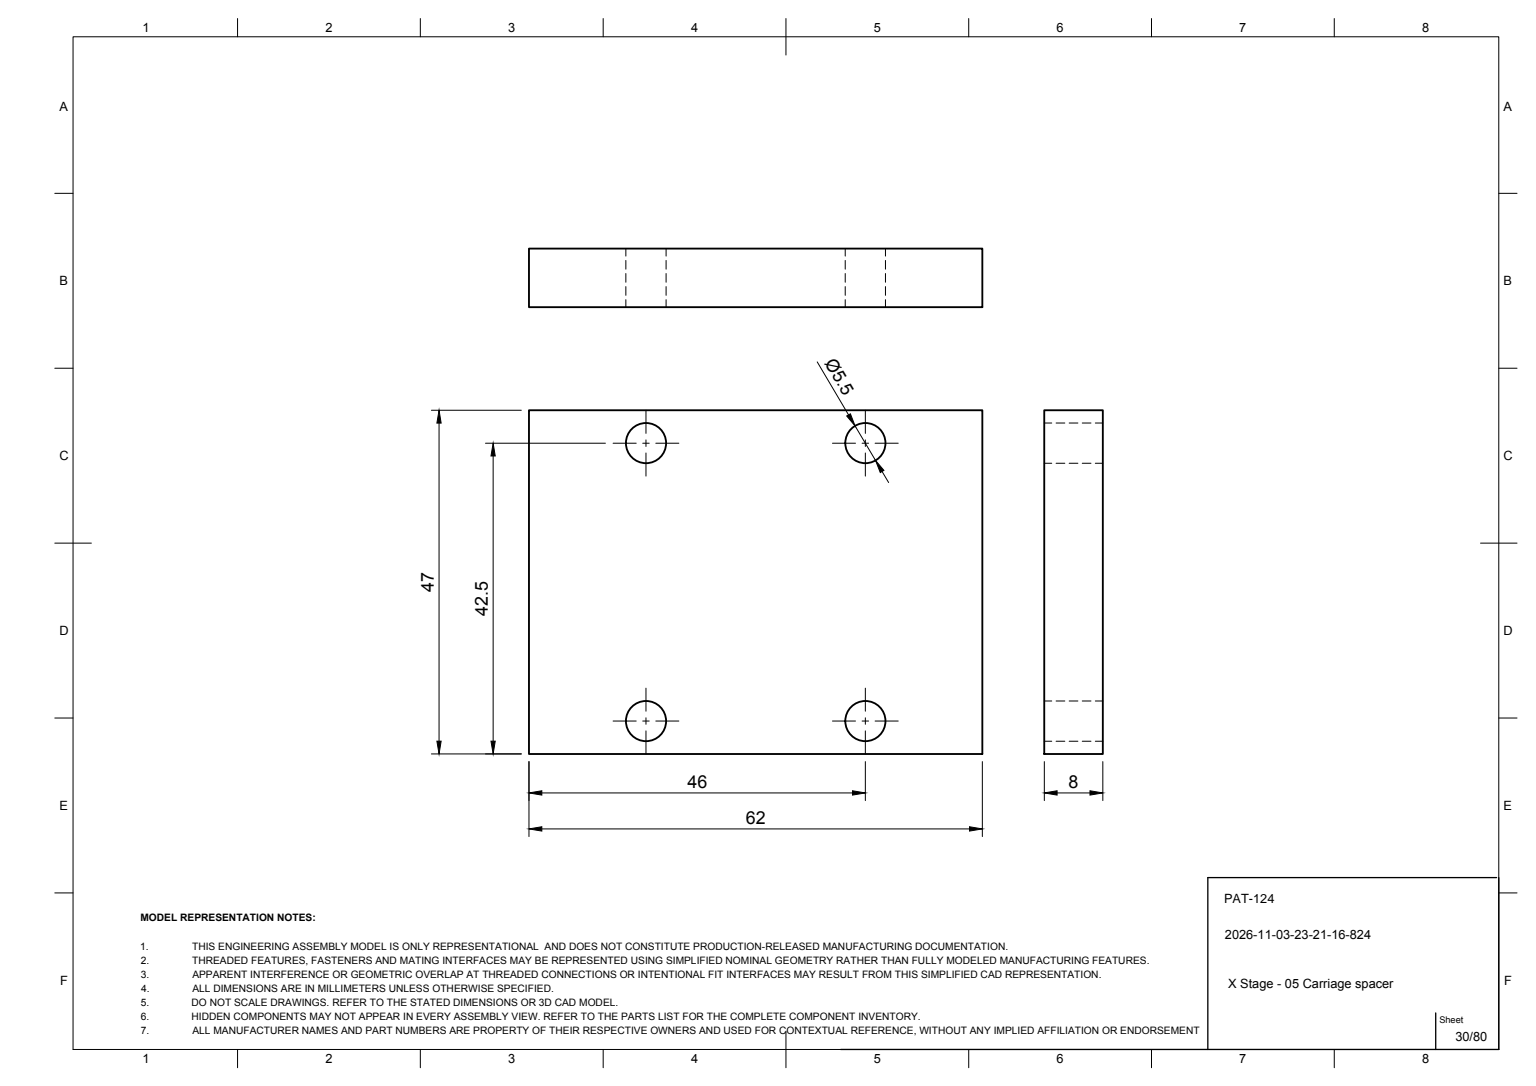
ISO-10303-21;
HEADER;
/* Generated by software containing ST-Developer
 * from STEP Tools, Inc. (www.steptools.com) 
 */

FILE_DESCRIPTION(
/* description */ ('XY cross-slide table'),
/* implementation_level */ '2;1');

FILE_NAME(
/* name */ 'X Stage - 05 Carriage spacer.step',
/* time_stamp */ '2026-10-28T03:22:46-07:00',
/* author */ (''),
/* organization */ (''),
/* preprocessor_version */ 'ST-DEVELOPER v20.2',
/* originating_system */ 'Autodesk Translation Framework v15.17.0.0',
/* authorisation */ '');

FILE_SCHEMA (('AUTOMOTIVE_DESIGN { 1 0 10303 214 3 1 1 }'));
ENDSEC;

DATA;
#10=MECHANICAL_DESIGN_GEOMETRIC_PRESENTATION_REPRESENTATION('',(#1706),#62984);
#1525=SHAPE_REPRESENTATION_RELATIONSHIP('SRR','None',#63376,#1608);
#1608=ADVANCED_BREP_SHAPE_REPRESENTATION('',(#1819),#62913);
#1706=STYLED_ITEM('',(#63898),#1819);
#1819=MANIFOLD_SOLID_BREP('Body1',#23000);
#2001=FACE_BOUND('',#4552,.T.);
#2002=FACE_BOUND('',#4553,.T.);
#2003=FACE_BOUND('',#4554,.T.);
#2004=FACE_BOUND('',#4555,.T.);
#2005=FACE_BOUND('',#4557,.T.);
#2006=FACE_BOUND('',#4558,.T.);
#2007=FACE_BOUND('',#4559,.T.);
#2008=FACE_BOUND('',#4560,.T.);
#2414=PLANE('',#24561);
#2415=PLANE('',#24562);
#2416=PLANE('',#24563);
#2417=PLANE('',#24564);
#2418=PLANE('',#24565);
#2419=PLANE('',#24566);
#3115=FACE_OUTER_BOUND('',#4543,.T.);
#3116=FACE_OUTER_BOUND('',#4544,.T.);
#3117=FACE_OUTER_BOUND('',#4545,.T.);
#3118=FACE_OUTER_BOUND('',#4546,.T.);
#3119=FACE_OUTER_BOUND('',#4547,.T.);
#3120=FACE_OUTER_BOUND('',#4548,.T.);
#3121=FACE_OUTER_BOUND('',#4549,.T.);
#3122=FACE_OUTER_BOUND('',#4550,.T.);
#3123=FACE_OUTER_BOUND('',#4551,.T.);
#3124=FACE_OUTER_BOUND('',#4556,.T.);
#4543=EDGE_LOOP('',(#15964,#15965,#15966,#15967));
#4544=EDGE_LOOP('',(#15968,#15969,#15970,#15971));
#4545=EDGE_LOOP('',(#15972,#15973,#15974,#15975));
#4546=EDGE_LOOP('',(#15976,#15977,#15978,#15979));
#4547=EDGE_LOOP('',(#15980,#15981,#15982,#15983));
#4548=EDGE_LOOP('',(#15984,#15985,#15986,#15987));
#4549=EDGE_LOOP('',(#15988,#15989,#15990,#15991));
#4550=EDGE_LOOP('',(#15992,#15993,#15994,#15995));
#4551=EDGE_LOOP('',(#15996,#15997,#15998,#15999));
#4552=EDGE_LOOP('',(#16000));
#4553=EDGE_LOOP('',(#16001));
#4554=EDGE_LOOP('',(#16002));
#4555=EDGE_LOOP('',(#16003));
#4556=EDGE_LOOP('',(#16004,#16005,#16006,#16007));
#4557=EDGE_LOOP('',(#16008));
#4558=EDGE_LOOP('',(#16009));
#4559=EDGE_LOOP('',(#16010));
#4560=EDGE_LOOP('',(#16011));
#6139=LINE('',#34688,#7626);
#6140=LINE('',#34694,#7627);
#6141=LINE('',#34700,#7628);
#6142=LINE('',#34706,#7629);
#6143=LINE('',#34711,#7630);
#6144=LINE('',#34713,#7631);
#6145=LINE('',#34715,#7632);
#6146=LINE('',#34716,#7633);
#6147=LINE('',#34719,#7634);
#6148=LINE('',#34721,#7635);
#6149=LINE('',#34722,#7636);
#6150=LINE('',#34725,#7637);
#6151=LINE('',#34727,#7638);
#6152=LINE('',#34728,#7639);
#6153=LINE('',#34730,#7640);
#6154=LINE('',#34731,#7641);
#7626=VECTOR('',#27796,0.275);
#7627=VECTOR('',#27803,0.275);
#7628=VECTOR('',#27810,0.275);
#7629=VECTOR('',#27817,0.275);
#7630=VECTOR('',#27822,1.);
#7631=VECTOR('',#27823,1.);
#7632=VECTOR('',#27824,1.);
#7633=VECTOR('',#27825,1.);
#7634=VECTOR('',#27828,1.);
#7635=VECTOR('',#27829,1.);
#7636=VECTOR('',#27830,1.);
#7637=VECTOR('',#27833,1.);
#7638=VECTOR('',#27834,1.);
#7639=VECTOR('',#27835,1.);
#7640=VECTOR('',#27838,1.);
#7641=VECTOR('',#27839,1.);
#9145=CIRCLE('',#24550,0.275);
#9146=CIRCLE('',#24551,0.275);
#9147=CIRCLE('',#24553,0.275);
#9148=CIRCLE('',#24554,0.275);
#9149=CIRCLE('',#24556,0.275);
#9150=CIRCLE('',#24557,0.275);
#9151=CIRCLE('',#24559,0.275);
#9152=CIRCLE('',#24560,0.275);
#10141=VERTEX_POINT('',#34685);
#10142=VERTEX_POINT('',#34687);
#10143=VERTEX_POINT('',#34691);
#10144=VERTEX_POINT('',#34693);
#10145=VERTEX_POINT('',#34697);
#10146=VERTEX_POINT('',#34699);
#10147=VERTEX_POINT('',#34703);
#10148=VERTEX_POINT('',#34705);
#10149=VERTEX_POINT('',#34709);
#10150=VERTEX_POINT('',#34710);
#10151=VERTEX_POINT('',#34712);
#10152=VERTEX_POINT('',#34714);
#10153=VERTEX_POINT('',#34718);
#10154=VERTEX_POINT('',#34720);
#10155=VERTEX_POINT('',#34724);
#10156=VERTEX_POINT('',#34726);
#12366=EDGE_CURVE('',#10141,#10141,#9145,.T.);
#12367=EDGE_CURVE('',#10141,#10142,#6139,.T.);
#12368=EDGE_CURVE('',#10142,#10142,#9146,.T.);
#12369=EDGE_CURVE('',#10143,#10143,#9147,.T.);
#12370=EDGE_CURVE('',#10143,#10144,#6140,.T.);
#12371=EDGE_CURVE('',#10144,#10144,#9148,.T.);
#12372=EDGE_CURVE('',#10145,#10145,#9149,.T.);
#12373=EDGE_CURVE('',#10145,#10146,#6141,.T.);
#12374=EDGE_CURVE('',#10146,#10146,#9150,.T.);
#12375=EDGE_CURVE('',#10147,#10147,#9151,.T.);
#12376=EDGE_CURVE('',#10147,#10148,#6142,.T.);
#12377=EDGE_CURVE('',#10148,#10148,#9152,.T.);
#12378=EDGE_CURVE('',#10149,#10150,#6143,.T.);
#12379=EDGE_CURVE('',#10150,#10151,#6144,.T.);
#12380=EDGE_CURVE('',#10152,#10151,#6145,.T.);
#12381=EDGE_CURVE('',#10149,#10152,#6146,.T.);
#12382=EDGE_CURVE('',#10153,#10149,#6147,.T.);
#12383=EDGE_CURVE('',#10154,#10152,#6148,.T.);
#12384=EDGE_CURVE('',#10153,#10154,#6149,.T.);
#12385=EDGE_CURVE('',#10155,#10153,#6150,.T.);
#12386=EDGE_CURVE('',#10156,#10154,#6151,.T.);
#12387=EDGE_CURVE('',#10155,#10156,#6152,.T.);
#12388=EDGE_CURVE('',#10150,#10155,#6153,.T.);
#12389=EDGE_CURVE('',#10151,#10156,#6154,.T.);
#15964=ORIENTED_EDGE('',*,*,#12366,.F.);
#15965=ORIENTED_EDGE('',*,*,#12367,.T.);
#15966=ORIENTED_EDGE('',*,*,#12368,.F.);
#15967=ORIENTED_EDGE('',*,*,#12367,.F.);
#15968=ORIENTED_EDGE('',*,*,#12369,.F.);
#15969=ORIENTED_EDGE('',*,*,#12370,.T.);
#15970=ORIENTED_EDGE('',*,*,#12371,.F.);
#15971=ORIENTED_EDGE('',*,*,#12370,.F.);
#15972=ORIENTED_EDGE('',*,*,#12372,.F.);
#15973=ORIENTED_EDGE('',*,*,#12373,.T.);
#15974=ORIENTED_EDGE('',*,*,#12374,.F.);
#15975=ORIENTED_EDGE('',*,*,#12373,.F.);
#15976=ORIENTED_EDGE('',*,*,#12375,.F.);
#15977=ORIENTED_EDGE('',*,*,#12376,.T.);
#15978=ORIENTED_EDGE('',*,*,#12377,.F.);
#15979=ORIENTED_EDGE('',*,*,#12376,.F.);
#15980=ORIENTED_EDGE('',*,*,#12378,.T.);
#15981=ORIENTED_EDGE('',*,*,#12379,.T.);
#15982=ORIENTED_EDGE('',*,*,#12380,.F.);
#15983=ORIENTED_EDGE('',*,*,#12381,.F.);
#15984=ORIENTED_EDGE('',*,*,#12382,.T.);
#15985=ORIENTED_EDGE('',*,*,#12381,.T.);
#15986=ORIENTED_EDGE('',*,*,#12383,.F.);
#15987=ORIENTED_EDGE('',*,*,#12384,.F.);
#15988=ORIENTED_EDGE('',*,*,#12385,.T.);
#15989=ORIENTED_EDGE('',*,*,#12384,.T.);
#15990=ORIENTED_EDGE('',*,*,#12386,.F.);
#15991=ORIENTED_EDGE('',*,*,#12387,.F.);
#15992=ORIENTED_EDGE('',*,*,#12388,.T.);
#15993=ORIENTED_EDGE('',*,*,#12387,.T.);
#15994=ORIENTED_EDGE('',*,*,#12389,.F.);
#15995=ORIENTED_EDGE('',*,*,#12379,.F.);
#15996=ORIENTED_EDGE('',*,*,#12389,.T.);
#15997=ORIENTED_EDGE('',*,*,#12386,.T.);
#15998=ORIENTED_EDGE('',*,*,#12383,.T.);
#15999=ORIENTED_EDGE('',*,*,#12380,.T.);
#16000=ORIENTED_EDGE('',*,*,#12368,.T.);
#16001=ORIENTED_EDGE('',*,*,#12371,.T.);
#16002=ORIENTED_EDGE('',*,*,#12374,.T.);
#16003=ORIENTED_EDGE('',*,*,#12377,.T.);
#16004=ORIENTED_EDGE('',*,*,#12388,.F.);
#16005=ORIENTED_EDGE('',*,*,#12378,.F.);
#16006=ORIENTED_EDGE('',*,*,#12382,.F.);
#16007=ORIENTED_EDGE('',*,*,#12385,.F.);
#16008=ORIENTED_EDGE('',*,*,#12366,.T.);
#16009=ORIENTED_EDGE('',*,*,#12369,.T.);
#16010=ORIENTED_EDGE('',*,*,#12372,.T.);
#16011=ORIENTED_EDGE('',*,*,#12375,.T.);
#21126=CYLINDRICAL_SURFACE('',#24549,0.275);
#21127=CYLINDRICAL_SURFACE('',#24552,0.275);
#21128=CYLINDRICAL_SURFACE('',#24555,0.275);
#21129=CYLINDRICAL_SURFACE('',#24558,0.275);
#21896=ADVANCED_FACE('',(#3115),#21126,.F.);
#21897=ADVANCED_FACE('',(#3116),#21127,.F.);
#21898=ADVANCED_FACE('',(#3117),#21128,.F.);
#21899=ADVANCED_FACE('',(#3118),#21129,.F.);
#21900=ADVANCED_FACE('',(#3119),#2414,.T.);
#21901=ADVANCED_FACE('',(#3120),#2415,.T.);
#21902=ADVANCED_FACE('',(#3121),#2416,.T.);
#21903=ADVANCED_FACE('',(#3122),#2417,.T.);
#21904=ADVANCED_FACE('',(#3123,#2001,#2002,#2003,#2004),#2418,.T.);
#21905=ADVANCED_FACE('',(#3124,#2005,#2006,#2007,#2008),#2419,.F.);
#23000=CLOSED_SHELL('',(#21896,#21897,#21898,#21899,#21900,#21901,#21902,
#21903,#21904,#21905));
#24548=AXIS2_PLACEMENT_3D('',#34683,#27790,#27791);
#24549=AXIS2_PLACEMENT_3D('',#34684,#27792,#27793);
#24550=AXIS2_PLACEMENT_3D('',#34686,#27794,#27795);
#24551=AXIS2_PLACEMENT_3D('',#34689,#27797,#27798);
#24552=AXIS2_PLACEMENT_3D('',#34690,#27799,#27800);
#24553=AXIS2_PLACEMENT_3D('',#34692,#27801,#27802);
#24554=AXIS2_PLACEMENT_3D('',#34695,#27804,#27805);
#24555=AXIS2_PLACEMENT_3D('',#34696,#27806,#27807);
#24556=AXIS2_PLACEMENT_3D('',#34698,#27808,#27809);
#24557=AXIS2_PLACEMENT_3D('',#34701,#27811,#27812);
#24558=AXIS2_PLACEMENT_3D('',#34702,#27813,#27814);
#24559=AXIS2_PLACEMENT_3D('',#34704,#27815,#27816);
#24560=AXIS2_PLACEMENT_3D('',#34707,#27818,#27819);
#24561=AXIS2_PLACEMENT_3D('',#34708,#27820,#27821);
#24562=AXIS2_PLACEMENT_3D('',#34717,#27826,#27827);
#24563=AXIS2_PLACEMENT_3D('',#34723,#27831,#27832);
#24564=AXIS2_PLACEMENT_3D('',#34729,#27836,#27837);
#24565=AXIS2_PLACEMENT_3D('',#34732,#27840,#27841);
#24566=AXIS2_PLACEMENT_3D('',#34733,#27842,#27843);
#27790=DIRECTION('axis',(0.,0.,1.));
#27791=DIRECTION('refdir',(1.,0.,0.));
#27792=DIRECTION('center_axis',(0.,0.,1.));
#27793=DIRECTION('ref_axis',(1.,0.,0.));
#27794=DIRECTION('center_axis',(0.,0.,1.));
#27795=DIRECTION('ref_axis',(1.,0.,0.));
#27796=DIRECTION('',(0.,0.,1.));
#27797=DIRECTION('center_axis',(0.,0.,-1.));
#27798=DIRECTION('ref_axis',(1.,0.,0.));
#27799=DIRECTION('center_axis',(0.,0.,1.));
#27800=DIRECTION('ref_axis',(1.,0.,0.));
#27801=DIRECTION('center_axis',(0.,0.,1.));
#27802=DIRECTION('ref_axis',(1.,0.,0.));
#27803=DIRECTION('',(0.,0.,1.));
#27804=DIRECTION('center_axis',(0.,0.,-1.));
#27805=DIRECTION('ref_axis',(1.,0.,0.));
#27806=DIRECTION('center_axis',(0.,0.,1.));
#27807=DIRECTION('ref_axis',(1.,0.,0.));
#27808=DIRECTION('center_axis',(0.,0.,1.));
#27809=DIRECTION('ref_axis',(1.,0.,0.));
#27810=DIRECTION('',(0.,0.,1.));
#27811=DIRECTION('center_axis',(0.,0.,-1.));
#27812=DIRECTION('ref_axis',(1.,0.,0.));
#27813=DIRECTION('center_axis',(0.,0.,1.));
#27814=DIRECTION('ref_axis',(1.,0.,0.));
#27815=DIRECTION('center_axis',(0.,0.,1.));
#27816=DIRECTION('ref_axis',(1.,0.,0.));
#27817=DIRECTION('',(0.,0.,1.));
#27818=DIRECTION('center_axis',(0.,0.,-1.));
#27819=DIRECTION('ref_axis',(1.,0.,0.));
#27820=DIRECTION('center_axis',(0.,1.,0.));
#27821=DIRECTION('ref_axis',(-1.,0.,0.));
#27822=DIRECTION('',(-1.,0.,0.));
#27823=DIRECTION('',(0.,0.,1.));
#27824=DIRECTION('',(-1.,0.,0.));
#27825=DIRECTION('',(0.,0.,1.));
#27826=DIRECTION('center_axis',(1.,0.,0.));
#27827=DIRECTION('ref_axis',(0.,1.,0.));
#27828=DIRECTION('',(0.,1.,0.));
#27829=DIRECTION('',(0.,1.,0.));
#27830=DIRECTION('',(0.,0.,1.));
#27831=DIRECTION('center_axis',(0.,-1.,0.));
#27832=DIRECTION('ref_axis',(1.,0.,0.));
#27833=DIRECTION('',(1.,0.,0.));
#27834=DIRECTION('',(1.,0.,0.));
#27835=DIRECTION('',(0.,0.,1.));
#27836=DIRECTION('center_axis',(-1.,0.,0.));
#27837=DIRECTION('ref_axis',(0.,-1.,0.));
#27838=DIRECTION('',(0.,-1.,0.));
#27839=DIRECTION('',(0.,-1.,0.));
#27840=DIRECTION('center_axis',(0.,0.,1.));
#27841=DIRECTION('ref_axis',(1.,0.,0.));
#27842=DIRECTION('center_axis',(0.,0.,1.));
#27843=DIRECTION('ref_axis',(1.,0.,0.));
#34683=CARTESIAN_POINT('',(0.,0.,0.));
#34684=CARTESIAN_POINT('Origin',(15.,-7.9,5.1));
#34685=CARTESIAN_POINT('',(14.725,-7.9,5.2));
#34686=CARTESIAN_POINT('Origin',(15.,-7.9,5.2));
#34687=CARTESIAN_POINT('',(14.725,-7.9,6.));
#34688=CARTESIAN_POINT('',(14.725,-7.9,5.1));
#34689=CARTESIAN_POINT('Origin',(15.,-7.9,6.));
#34690=CARTESIAN_POINT('Origin',(12.,-4.1,5.1));
#34691=CARTESIAN_POINT('',(11.725,-4.1,5.2));
#34692=CARTESIAN_POINT('Origin',(12.,-4.1,5.2));
#34693=CARTESIAN_POINT('',(11.725,-4.1,6.));
#34694=CARTESIAN_POINT('',(11.725,-4.1,5.1));
#34695=CARTESIAN_POINT('Origin',(12.,-4.1,6.));
#34696=CARTESIAN_POINT('Origin',(12.,-7.9,5.1));
#34697=CARTESIAN_POINT('',(11.725,-7.9,5.2));
#34698=CARTESIAN_POINT('Origin',(12.,-7.9,5.2));
#34699=CARTESIAN_POINT('',(11.725,-7.9,6.));
#34700=CARTESIAN_POINT('',(11.725,-7.9,5.1));
#34701=CARTESIAN_POINT('Origin',(12.,-7.9,6.));
#34702=CARTESIAN_POINT('Origin',(15.,-4.1,5.1));
#34703=CARTESIAN_POINT('',(14.725,-4.1,5.2));
#34704=CARTESIAN_POINT('Origin',(15.,-4.1,5.2));
#34705=CARTESIAN_POINT('',(14.725,-4.1,6.));
#34706=CARTESIAN_POINT('',(14.725,-4.1,5.1));
#34707=CARTESIAN_POINT('Origin',(15.,-4.1,6.));
#34708=CARTESIAN_POINT('Origin',(16.6,-3.65,5.2));
#34709=CARTESIAN_POINT('',(16.6,-3.65,5.2));
#34710=CARTESIAN_POINT('',(10.4,-3.65,5.2));
#34711=CARTESIAN_POINT('',(16.6,-3.65,5.2));
#34712=CARTESIAN_POINT('',(10.4,-3.65,6.));
#34713=CARTESIAN_POINT('',(10.4,-3.65,5.2));
#34714=CARTESIAN_POINT('',(16.6,-3.65,6.));
#34715=CARTESIAN_POINT('',(16.6,-3.65,6.));
#34716=CARTESIAN_POINT('',(16.6,-3.65,5.2));
#34717=CARTESIAN_POINT('Origin',(16.6,-8.35,5.2));
#34718=CARTESIAN_POINT('',(16.6,-8.35,5.2));
#34719=CARTESIAN_POINT('',(16.6,-8.35,5.2));
#34720=CARTESIAN_POINT('',(16.6,-8.35,6.));
#34721=CARTESIAN_POINT('',(16.6,-8.35,6.));
#34722=CARTESIAN_POINT('',(16.6,-8.35,5.2));
#34723=CARTESIAN_POINT('Origin',(10.4,-8.35,5.2));
#34724=CARTESIAN_POINT('',(10.4,-8.35,5.2));
#34725=CARTESIAN_POINT('',(10.4,-8.35,5.2));
#34726=CARTESIAN_POINT('',(10.4,-8.35,6.));
#34727=CARTESIAN_POINT('',(10.4,-8.35,6.));
#34728=CARTESIAN_POINT('',(10.4,-8.35,5.2));
#34729=CARTESIAN_POINT('Origin',(10.4,-3.65,5.2));
#34730=CARTESIAN_POINT('',(10.4,-3.65,5.2));
#34731=CARTESIAN_POINT('',(10.4,-3.65,6.));
#34732=CARTESIAN_POINT('Origin',(13.5,-6.,6.));
#34733=CARTESIAN_POINT('Origin',(13.5,-6.,5.2));
#62814=UNCERTAINTY_MEASURE_WITH_UNIT(LENGTH_MEASURE(0.001),#62985,
'DISTANCE_ACCURACY_VALUE',
'Maximum model space distance between geometric entities at asserted c
onnectivities');
#62885=UNCERTAINTY_MEASURE_WITH_UNIT(LENGTH_MEASURE(0.001),#62985,
'DISTANCE_ACCURACY_VALUE',
'Maximum model space distance between geometric entities at asserted c
onnectivities');
#62913=(
GEOMETRIC_REPRESENTATION_CONTEXT(3)
GLOBAL_UNCERTAINTY_ASSIGNED_CONTEXT((#62814))
GLOBAL_UNIT_ASSIGNED_CONTEXT((#62985,#62987,#62988))
REPRESENTATION_CONTEXT('','3D')
);
#62984=(
GEOMETRIC_REPRESENTATION_CONTEXT(3)
GLOBAL_UNCERTAINTY_ASSIGNED_CONTEXT((#62885))
GLOBAL_UNIT_ASSIGNED_CONTEXT((#62985,#62987,#62988))
REPRESENTATION_CONTEXT('','3D')
);
#62985=(
LENGTH_UNIT()
NAMED_UNIT(*)
SI_UNIT(.CENTI.,.METRE.)
);
#62987=(
NAMED_UNIT(*)
PLANE_ANGLE_UNIT()
SI_UNIT($,.RADIAN.)
);
#62988=(
NAMED_UNIT(*)
SI_UNIT($,.STERADIAN.)
SOLID_ANGLE_UNIT()
);
#63016=SHAPE_DEFINITION_REPRESENTATION(#63124,#63376);
#63124=PRODUCT_DEFINITION_SHAPE('',$,#63475);
#63376=SHAPE_REPRESENTATION('',(#24548),#62913);
#63447=PRODUCT_DEFINITION_CONTEXT('part definition',#63743,'design');
#63475=PRODUCT_DEFINITION('X Stage - 05 Carriage spacer',
'X Stage - 05 Carriage spacer',#63573,#63447);
#63573=PRODUCT_DEFINITION_FORMATION('',$,#63772);
#63743=APPLICATION_CONTEXT(
'Core Data for Automotive Mechanical Design Process');
#63744=PRODUCT_CONTEXT('part definition',#63743,'mechanical');
#63772=PRODUCT('X Stage - 05 Carriage spacer',
'X Stage - 05 Carriage spacer','X Stage - 05 Carriage spacer',(#63744));
#63892=COLOUR_RGB('Light Blue',0.38,0.62,0.78);
#63893=FILL_AREA_STYLE_COLOUR('',#63892);
#63894=FILL_AREA_STYLE('',(#63893));
#63895=SURFACE_STYLE_FILL_AREA(#63894);
#63896=SURFACE_SIDE_STYLE('',(#63895));
#63897=SURFACE_STYLE_USAGE(.BOTH.,#63896);
#63898=PRESENTATION_STYLE_ASSIGNMENT((#63897));
ENDSEC;
END-ISO-10303-21;
